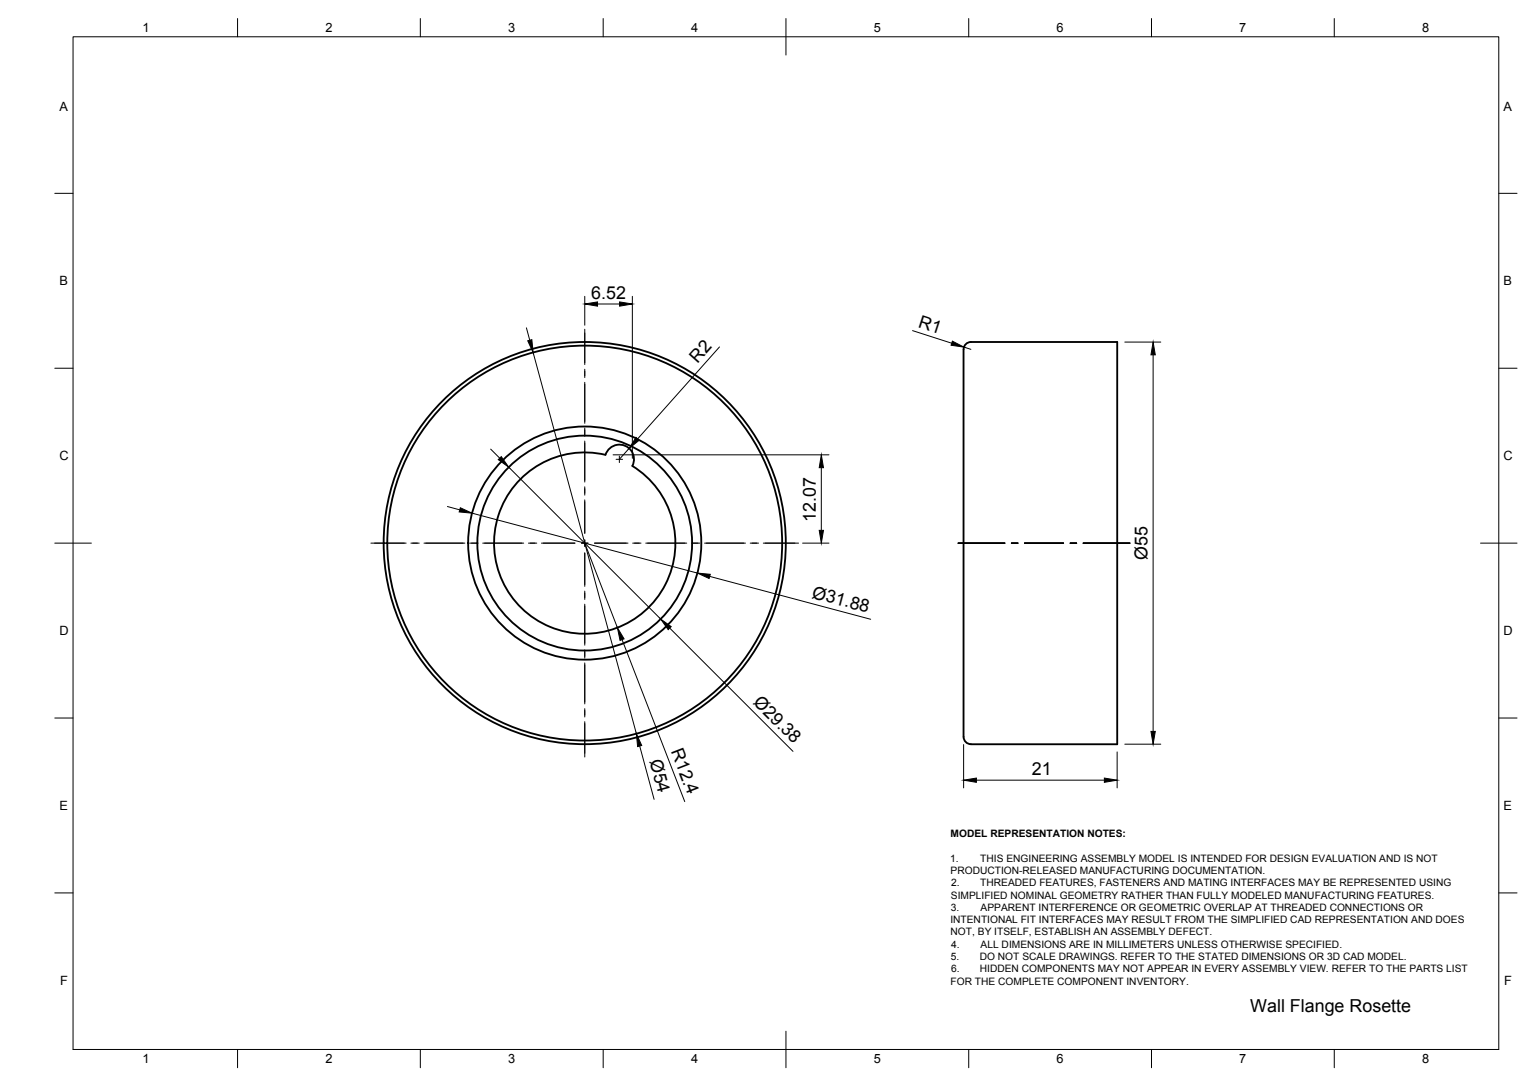
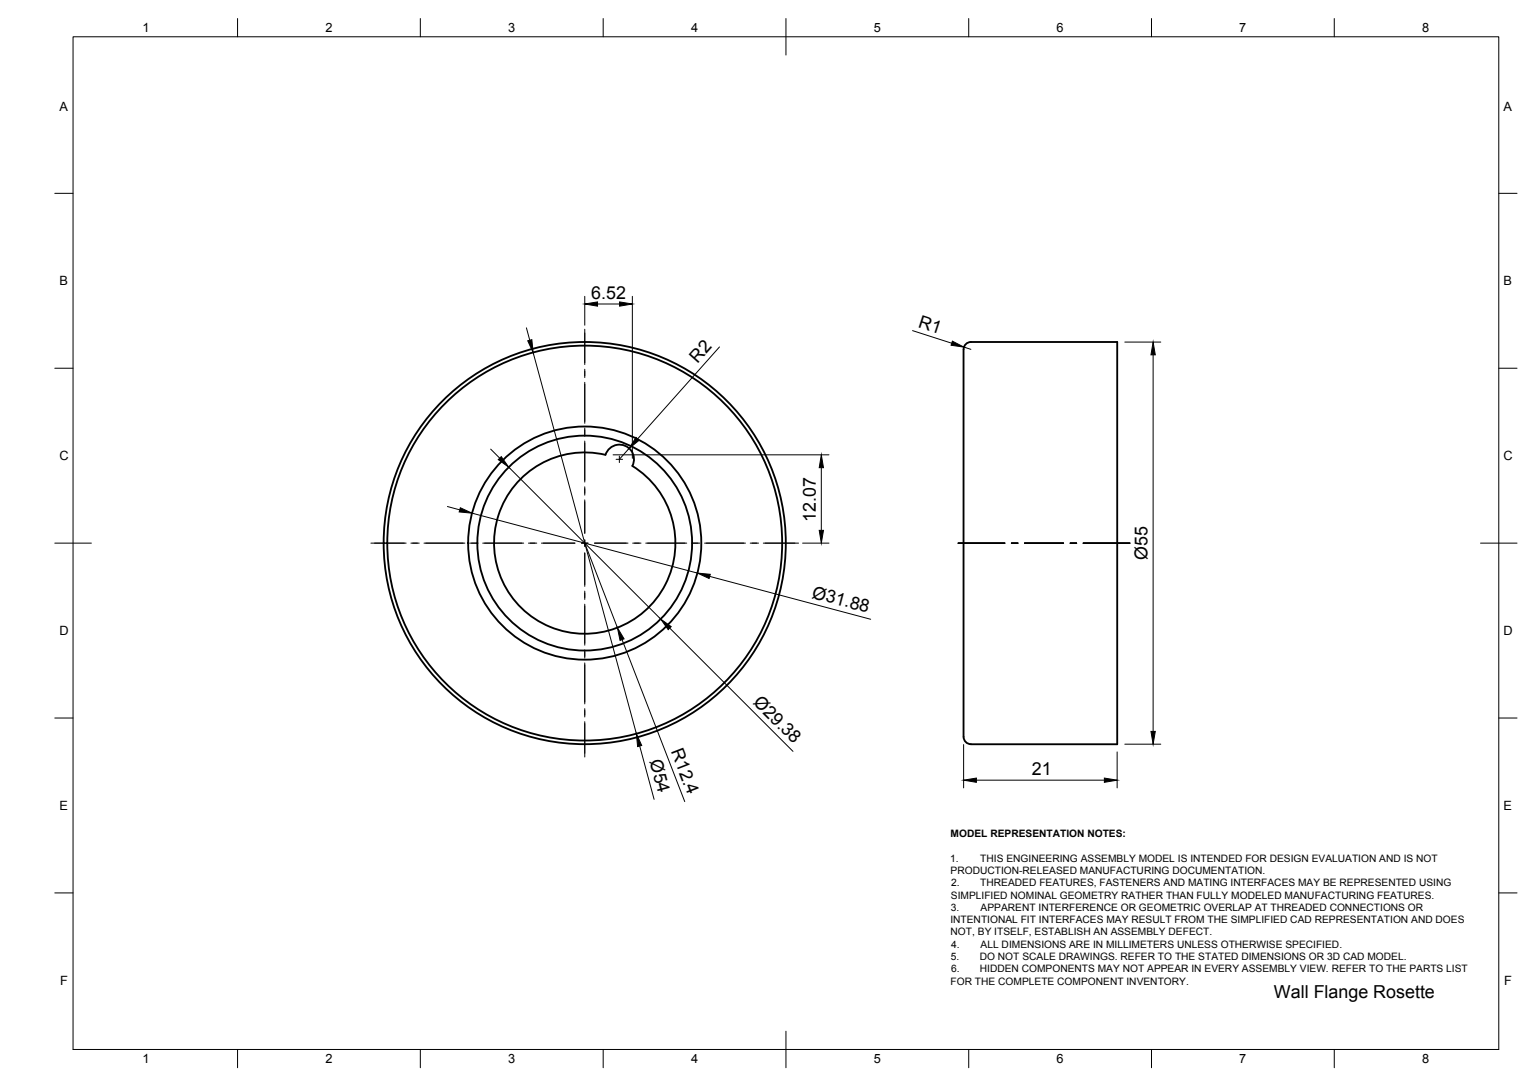
ISO-10303-21;
HEADER;
/* Generated by software containing ST-Developer
 * from STEP Tools, Inc. (www.steptools.com) 
 */

FILE_DESCRIPTION(
/* description */ ('STEP AP214'),
/* implementation_level */ '2;1');

FILE_NAME(
/* name */ 'Wall Flange Rosette.step',
/* time_stamp */ '2026-10-05T23:18:41-07:00',
/* author */ (''),
/* organization */ (''),
/* preprocessor_version */ 'ST-DEVELOPER v20.2',
/* originating_system */ 'Autodesk Translation Framework v15.15.0.0',
/* authorisation */ '');

FILE_SCHEMA (('AUTOMOTIVE_DESIGN { 1 0 10303 214 3 1 1 }'));
ENDSEC;

DATA;
#10=MECHANICAL_DESIGN_GEOMETRIC_PRESENTATION_REPRESENTATION('',(#106),#221662);
#68=MANIFOLD_SOLID_BREP('Body1',#79328);
#80=SHAPE_REPRESENTATION_RELATIONSHIP('SRR','None',#221715,#93);
#93=ADVANCED_BREP_SHAPE_REPRESENTATION('',(#68),#221655);
#106=STYLED_ITEM('',(#221783),#68);
#297=FACE_BOUND('',#24816,.T.);
#298=FACE_BOUND('',#24818,.T.);
#299=FACE_BOUND('',#24820,.T.);
#300=FACE_BOUND('',#24823,.T.);
#301=FACE_BOUND('',#24825,.T.);
#1896=TOROIDAL_SURFACE('',#80767,26.5,1.);
#1897=TOROIDAL_SURFACE('',#80779,26.5,0.5);
#1942=CONICAL_SURFACE('',#80785,15.31367390024,0.849141474959914);
#1943=CONICAL_SURFACE('',#80792,15.125,0.849141474959914);
#2233=CYLINDRICAL_SURFACE('',#80771,27.5);
#2234=CYLINDRICAL_SURFACE('',#80773,12.4);
#2235=CYLINDRICAL_SURFACE('',#80776,2.00000000000001);
#2236=CYLINDRICAL_SURFACE('',#80783,27.);
#3153=LINE('',#177954,#10220);
#3154=LINE('',#177961,#10221);
#3155=LINE('',#177964,#10222);
#3156=LINE('',#177977,#10223);
#3157=LINE('',#177982,#10224);
#3158=LINE('',#177991,#10225);
#10220=VECTOR('',#89196,27.5);
#10221=VECTOR('',#89203,1000.);
#10222=VECTOR('',#89206,1000.);
#10223=VECTOR('',#89225,27.);
#10224=VECTOR('',#89230,15.31367390024);
#10225=VECTOR('',#89243,15.125);
#16989=PLANE('',#80788);
#16990=PLANE('',#80789);
#16991=PLANE('',#80790);
#16992=PLANE('',#80794);
#16993=PLANE('',#80795);
#20741=FACE_OUTER_BOUND('',#24808,.T.);
#20742=FACE_OUTER_BOUND('',#24809,.T.);
#20743=FACE_OUTER_BOUND('',#24810,.T.);
#20744=FACE_OUTER_BOUND('',#24811,.T.);
#20745=FACE_OUTER_BOUND('',#24812,.T.);
#20746=FACE_OUTER_BOUND('',#24813,.T.);
#20747=FACE_OUTER_BOUND('',#24814,.T.);
#20748=FACE_OUTER_BOUND('',#24815,.T.);
#20749=FACE_OUTER_BOUND('',#24817,.T.);
#20750=FACE_OUTER_BOUND('',#24819,.T.);
#20751=FACE_OUTER_BOUND('',#24821,.T.);
#20752=FACE_OUTER_BOUND('',#24822,.T.);
#20753=FACE_OUTER_BOUND('',#24824,.T.);
#24808=EDGE_LOOP('',(#56653,#56654,#56655,#56656));
#24809=EDGE_LOOP('',(#56657,#56658,#56659,#56660));
#24810=EDGE_LOOP('',(#56661,#56662,#56663,#56664));
#24811=EDGE_LOOP('',(#56665,#56666,#56667,#56668));
#24812=EDGE_LOOP('',(#56669,#56670,#56671,#56672));
#24813=EDGE_LOOP('',(#56673,#56674,#56675,#56676));
#24814=EDGE_LOOP('',(#56677,#56678,#56679,#56680));
#24815=EDGE_LOOP('',(#56681));
#24816=EDGE_LOOP('',(#56682));
#24817=EDGE_LOOP('',(#56683));
#24818=EDGE_LOOP('',(#56684,#56685));
#24819=EDGE_LOOP('',(#56686));
#24820=EDGE_LOOP('',(#56687,#56688));
#24821=EDGE_LOOP('',(#56689,#56690,#56691,#56692));
#24822=EDGE_LOOP('',(#56693));
#24823=EDGE_LOOP('',(#56694));
#24824=EDGE_LOOP('',(#56695));
#24825=EDGE_LOOP('',(#56696));
#31299=CIRCLE('',#80768,26.49999955823);
#31300=CIRCLE('',#80769,1.);
#31301=CIRCLE('',#80770,27.5);
#31302=CIRCLE('',#80772,27.5);
#31303=CIRCLE('',#80774,12.4);
#31304=CIRCLE('',#80775,12.4);
#31305=CIRCLE('',#80777,2.);
#31306=CIRCLE('',#80778,2.);
#31307=CIRCLE('',#80780,27.);
#31308=CIRCLE('',#80781,0.5);
#31309=CIRCLE('',#80782,26.5);
#31310=CIRCLE('',#80784,27.);
#31311=CIRCLE('',#80786,15.93867390024);
#31312=CIRCLE('',#80787,14.68867390024);
#31313=CIRCLE('',#80791,14.5);
#31314=CIRCLE('',#80793,15.75);
#34858=VERTEX_POINT('',#177947);
#34859=VERTEX_POINT('',#177949);
#34860=VERTEX_POINT('',#177953);
#34861=VERTEX_POINT('',#177957);
#34862=VERTEX_POINT('',#177958);
#34863=VERTEX_POINT('',#177960);
#34864=VERTEX_POINT('',#177962);
#34865=VERTEX_POINT('',#177969);
#34866=VERTEX_POINT('',#177971);
#34867=VERTEX_POINT('',#177975);
#34868=VERTEX_POINT('',#177979);
#34869=VERTEX_POINT('',#177981);
#34870=VERTEX_POINT('',#177987);
#34871=VERTEX_POINT('',#177990);
#43159=EDGE_CURVE('',#34858,#34858,#31299,.T.);
#43160=EDGE_CURVE('',#34858,#34859,#31300,.T.);
#43161=EDGE_CURVE('',#34859,#34859,#31301,.T.);
#43162=EDGE_CURVE('',#34859,#34860,#3153,.T.);
#43163=EDGE_CURVE('',#34860,#34860,#31302,.T.);
#43164=EDGE_CURVE('',#34861,#34862,#31303,.T.);
#43165=EDGE_CURVE('',#34863,#34861,#3154,.T.);
#43166=EDGE_CURVE('',#34863,#34864,#31304,.T.);
#43167=EDGE_CURVE('',#34864,#34862,#3155,.T.);
#43168=EDGE_CURVE('',#34862,#34861,#31305,.T.);
#43169=EDGE_CURVE('',#34864,#34863,#31306,.T.);
#43170=EDGE_CURVE('',#34865,#34865,#31307,.T.);
#43171=EDGE_CURVE('',#34865,#34866,#31308,.T.);
#43172=EDGE_CURVE('',#34866,#34866,#31309,.T.);
#43173=EDGE_CURVE('',#34867,#34867,#31310,.T.);
#43174=EDGE_CURVE('',#34867,#34865,#3156,.T.);
#43175=EDGE_CURVE('',#34868,#34868,#31311,.T.);
#43176=EDGE_CURVE('',#34868,#34869,#3157,.T.);
#43177=EDGE_CURVE('',#34869,#34869,#31312,.T.);
#43178=EDGE_CURVE('',#34870,#34870,#31313,.T.);
#43179=EDGE_CURVE('',#34870,#34871,#3158,.T.);
#43180=EDGE_CURVE('',#34871,#34871,#31314,.T.);
#56653=ORIENTED_EDGE('',*,*,#43159,.F.);
#56654=ORIENTED_EDGE('',*,*,#43160,.T.);
#56655=ORIENTED_EDGE('',*,*,#43161,.T.);
#56656=ORIENTED_EDGE('',*,*,#43160,.F.);
#56657=ORIENTED_EDGE('',*,*,#43161,.F.);
#56658=ORIENTED_EDGE('',*,*,#43162,.T.);
#56659=ORIENTED_EDGE('',*,*,#43163,.T.);
#56660=ORIENTED_EDGE('',*,*,#43162,.F.);
#56661=ORIENTED_EDGE('',*,*,#43164,.F.);
#56662=ORIENTED_EDGE('',*,*,#43165,.F.);
#56663=ORIENTED_EDGE('',*,*,#43166,.T.);
#56664=ORIENTED_EDGE('',*,*,#43167,.T.);
#56665=ORIENTED_EDGE('',*,*,#43168,.F.);
#56666=ORIENTED_EDGE('',*,*,#43167,.F.);
#56667=ORIENTED_EDGE('',*,*,#43169,.T.);
#56668=ORIENTED_EDGE('',*,*,#43165,.T.);
#56669=ORIENTED_EDGE('',*,*,#43170,.F.);
#56670=ORIENTED_EDGE('',*,*,#43171,.T.);
#56671=ORIENTED_EDGE('',*,*,#43172,.T.);
#56672=ORIENTED_EDGE('',*,*,#43171,.F.);
#56673=ORIENTED_EDGE('',*,*,#43173,.F.);
#56674=ORIENTED_EDGE('',*,*,#43174,.T.);
#56675=ORIENTED_EDGE('',*,*,#43170,.T.);
#56676=ORIENTED_EDGE('',*,*,#43174,.F.);
#56677=ORIENTED_EDGE('',*,*,#43175,.F.);
#56678=ORIENTED_EDGE('',*,*,#43176,.T.);
#56679=ORIENTED_EDGE('',*,*,#43177,.T.);
#56680=ORIENTED_EDGE('',*,*,#43176,.F.);
#56681=ORIENTED_EDGE('',*,*,#43172,.F.);
#56682=ORIENTED_EDGE('',*,*,#43175,.T.);
#56683=ORIENTED_EDGE('',*,*,#43177,.F.);
#56684=ORIENTED_EDGE('',*,*,#43169,.F.);
#56685=ORIENTED_EDGE('',*,*,#43166,.F.);
#56686=ORIENTED_EDGE('',*,*,#43178,.T.);
#56687=ORIENTED_EDGE('',*,*,#43168,.T.);
#56688=ORIENTED_EDGE('',*,*,#43164,.T.);
#56689=ORIENTED_EDGE('',*,*,#43178,.F.);
#56690=ORIENTED_EDGE('',*,*,#43179,.T.);
#56691=ORIENTED_EDGE('',*,*,#43180,.T.);
#56692=ORIENTED_EDGE('',*,*,#43179,.F.);
#56693=ORIENTED_EDGE('',*,*,#43159,.T.);
#56694=ORIENTED_EDGE('',*,*,#43180,.F.);
#56695=ORIENTED_EDGE('',*,*,#43163,.F.);
#56696=ORIENTED_EDGE('',*,*,#43173,.T.);
#76171=ADVANCED_FACE('',(#20741),#1896,.T.);
#76172=ADVANCED_FACE('',(#20742),#2233,.T.);
#76173=ADVANCED_FACE('',(#20743),#2234,.F.);
#76174=ADVANCED_FACE('',(#20744),#2235,.F.);
#76175=ADVANCED_FACE('',(#20745),#1897,.F.);
#76176=ADVANCED_FACE('',(#20746),#2236,.F.);
#76177=ADVANCED_FACE('',(#20747),#1942,.T.);
#76178=ADVANCED_FACE('',(#20748,#297),#16989,.F.);
#76179=ADVANCED_FACE('',(#20749,#298),#16990,.F.);
#76180=ADVANCED_FACE('',(#20750,#299),#16991,.T.);
#76181=ADVANCED_FACE('',(#20751),#1943,.F.);
#76182=ADVANCED_FACE('',(#20752,#300),#16992,.T.);
#76183=ADVANCED_FACE('',(#20753,#301),#16993,.F.);
#79328=CLOSED_SHELL('',(#76171,#76172,#76173,#76174,#76175,#76176,#76177,
#76178,#76179,#76180,#76181,#76182,#76183));
#80766=AXIS2_PLACEMENT_3D('',#177945,#89184,#89185);
#80767=AXIS2_PLACEMENT_3D('',#177946,#89186,#89187);
#80768=AXIS2_PLACEMENT_3D('',#177948,#89188,#89189);
#80769=AXIS2_PLACEMENT_3D('',#177950,#89190,#89191);
#80770=AXIS2_PLACEMENT_3D('',#177951,#89192,#89193);
#80771=AXIS2_PLACEMENT_3D('',#177952,#89194,#89195);
#80772=AXIS2_PLACEMENT_3D('',#177955,#89197,#89198);
#80773=AXIS2_PLACEMENT_3D('',#177956,#89199,#89200);
#80774=AXIS2_PLACEMENT_3D('',#177959,#89201,#89202);
#80775=AXIS2_PLACEMENT_3D('',#177963,#89204,#89205);
#80776=AXIS2_PLACEMENT_3D('',#177965,#89207,#89208);
#80777=AXIS2_PLACEMENT_3D('',#177966,#89209,#89210);
#80778=AXIS2_PLACEMENT_3D('',#177967,#89211,#89212);
#80779=AXIS2_PLACEMENT_3D('',#177968,#89213,#89214);
#80780=AXIS2_PLACEMENT_3D('',#177970,#89215,#89216);
#80781=AXIS2_PLACEMENT_3D('',#177972,#89217,#89218);
#80782=AXIS2_PLACEMENT_3D('',#177973,#89219,#89220);
#80783=AXIS2_PLACEMENT_3D('',#177974,#89221,#89222);
#80784=AXIS2_PLACEMENT_3D('',#177976,#89223,#89224);
#80785=AXIS2_PLACEMENT_3D('',#177978,#89226,#89227);
#80786=AXIS2_PLACEMENT_3D('',#177980,#89228,#89229);
#80787=AXIS2_PLACEMENT_3D('',#177983,#89231,#89232);
#80788=AXIS2_PLACEMENT_3D('',#177984,#89233,#89234);
#80789=AXIS2_PLACEMENT_3D('',#177985,#89235,#89236);
#80790=AXIS2_PLACEMENT_3D('',#177986,#89237,#89238);
#80791=AXIS2_PLACEMENT_3D('',#177988,#89239,#89240);
#80792=AXIS2_PLACEMENT_3D('',#177989,#89241,#89242);
#80793=AXIS2_PLACEMENT_3D('',#177992,#89244,#89245);
#80794=AXIS2_PLACEMENT_3D('',#177993,#89246,#89247);
#80795=AXIS2_PLACEMENT_3D('',#177994,#89248,#89249);
#89184=DIRECTION('axis',(0.,0.,1.));
#89185=DIRECTION('refdir',(1.,0.,0.));
#89186=DIRECTION('center_axis',(1.,0.,0.));
#89187=DIRECTION('ref_axis',(0.,0.924224592736303,0.381849318686593));
#89188=DIRECTION('center_axis',(1.,0.,0.));
#89189=DIRECTION('ref_axis',(0.,0.381849318686592,-0.924224592736303));
#89190=DIRECTION('center_axis',(0.,0.381849318686593,-0.924224592736303));
#89191=DIRECTION('ref_axis',(0.,-0.924224592736303,-0.381849318686593));
#89192=DIRECTION('center_axis',(1.,0.,0.));
#89193=DIRECTION('ref_axis',(0.,0.381849318686593,-0.924224592736303));
#89194=DIRECTION('center_axis',(1.,0.,0.));
#89195=DIRECTION('ref_axis',(0.,0.924224592736303,0.381849318686593));
#89196=DIRECTION('',(-1.,0.,0.));
#89197=DIRECTION('center_axis',(1.,0.,0.));
#89198=DIRECTION('ref_axis',(0.,0.381849318686593,-0.924224592736303));
#89199=DIRECTION('center_axis',(-1.,0.,0.));
#89200=DIRECTION('ref_axis',(0.,0.381849318686589,-0.924224592736304));
#89201=DIRECTION('center_axis',(-1.,0.,0.));
#89202=DIRECTION('ref_axis',(0.,-0.228299548172813,0.973590938897897));
#89203=DIRECTION('',(1.,0.,0.));
#89204=DIRECTION('center_axis',(-1.,0.,0.));
#89205=DIRECTION('ref_axis',(0.,-0.228299548172813,0.973590938897897));
#89206=DIRECTION('',(1.,0.,0.));
#89207=DIRECTION('center_axis',(-1.,0.,0.));
#89208=DIRECTION('ref_axis',(0.,-0.381849318686606,0.924224592736298));
#89209=DIRECTION('center_axis',(-1.,0.,0.));
#89210=DIRECTION('ref_axis',(0.,-0.890419977397047,-0.455139828901232));
#89211=DIRECTION('center_axis',(-1.,0.,0.));
#89212=DIRECTION('ref_axis',(0.,-0.890419977397047,-0.455139828901232));
#89213=DIRECTION('center_axis',(1.,0.,0.));
#89214=DIRECTION('ref_axis',(0.,0.924224592736303,0.381849318686593));
#89215=DIRECTION('center_axis',(1.,0.,0.));
#89216=DIRECTION('ref_axis',(0.,0.381849318686593,-0.924224592736303));
#89217=DIRECTION('center_axis',(0.,-0.381849318686593,0.924224592736303));
#89218=DIRECTION('ref_axis',(0.,-0.924224592736303,-0.381849318686593));
#89219=DIRECTION('center_axis',(1.,0.,0.));
#89220=DIRECTION('ref_axis',(0.,0.381849318686592,-0.924224592736303));
#89221=DIRECTION('center_axis',(1.,0.,0.));
#89222=DIRECTION('ref_axis',(0.,0.924224592736303,0.381849318686593));
#89223=DIRECTION('center_axis',(1.,0.,0.));
#89224=DIRECTION('ref_axis',(0.,0.381849318686593,-0.924224592736303));
#89225=DIRECTION('',(1.,0.,0.));
#89226=DIRECTION('center_axis',(1.,2.78424187714042E-18,1.15032739033389E-18));
#89227=DIRECTION('ref_axis',(-3.01251654524499E-18,0.924224592736303,0.381849318686592));
#89228=DIRECTION('center_axis',(1.,0.,0.));
#89229=DIRECTION('ref_axis',(0.,-0.924224592736303,-0.381849318686593));
#89230=DIRECTION('',(-0.660627895620383,0.693827893847185,0.286659444721021));
#89231=DIRECTION('center_axis',(1.,0.,0.));
#89232=DIRECTION('ref_axis',(0.,0.924224592736303,0.381849318686593));
#89233=DIRECTION('center_axis',(1.,0.,0.));
#89234=DIRECTION('ref_axis',(0.,1.,0.));
#89235=DIRECTION('center_axis',(1.,0.,0.));
#89236=DIRECTION('ref_axis',(0.,1.,0.));
#89237=DIRECTION('center_axis',(1.,0.,0.));
#89238=DIRECTION('ref_axis',(0.,1.,0.));
#89239=DIRECTION('center_axis',(1.,0.,0.));
#89240=DIRECTION('ref_axis',(0.,0.924224592736303,0.381849318686593));
#89241=DIRECTION('center_axis',(1.,-4.17704712177877E-17,-1.72577381094218E-17));
#89242=DIRECTION('ref_axis',(4.51951522888177E-17,0.924224592736303,0.381849318686593));
#89243=DIRECTION('',(0.660627895620383,-0.693827893847184,-0.286659444721022));
#89244=DIRECTION('center_axis',(1.,0.,0.));
#89245=DIRECTION('ref_axis',(0.,0.924224592736303,0.381849318686592));
#89246=DIRECTION('center_axis',(1.,0.,0.));
#89247=DIRECTION('ref_axis',(0.,1.,0.));
#89248=DIRECTION('center_axis',(1.,0.,0.));
#89249=DIRECTION('ref_axis',(0.,1.,0.));
#177945=CARTESIAN_POINT('',(0.,0.,0.));
#177946=CARTESIAN_POINT('Origin',(-30.5675364832709,75.,72.98888938658));
#177947=CARTESIAN_POINT('',(-29.5675364832709,50.5080487007827,62.8698826100749));
#177948=CARTESIAN_POINT('Origin',(-29.5675364832709,75.,72.98888938658));
#177949=CARTESIAN_POINT('',(-30.5675364832709,49.5838236997517,62.4880331226987));
#177950=CARTESIAN_POINT('Origin',(-30.5675364832709,50.508048292488,62.8698824413853));
#177951=CARTESIAN_POINT('Origin',(-30.5675364832709,75.,72.98888938658));
#177952=CARTESIAN_POINT('Origin',(-50.5675364832709,75.,72.98888938658));
#177953=CARTESIAN_POINT('',(-50.5675364832709,49.5838236997517,62.4880331226987));
#177954=CARTESIAN_POINT('',(-50.5675364832709,49.5838236997517,62.4880331226987));
#177955=CARTESIAN_POINT('Origin',(-50.5675364832709,75.,72.98888938658));
#177956=CARTESIAN_POINT('Origin',(-50.5675364832709,75.,72.98888938658));
#177957=CARTESIAN_POINT('',(-30.6675364832709,72.1690856026562,85.0614170289144));
#177958=CARTESIAN_POINT('',(-30.6675364832709,68.4842284934922,83.5389946787084));
#177959=CARTESIAN_POINT('Origin',(-30.6675364832709,75.,72.98888938658));
#177960=CARTESIAN_POINT('',(-31.1675364832709,72.1690856026562,85.0614170289144));
#177961=CARTESIAN_POINT('',(-31.1675364832709,72.1690856026562,85.0614170289144));
#177962=CARTESIAN_POINT('',(-31.1675364832709,68.4842284934922,83.5389946787084));
#177963=CARTESIAN_POINT('Origin',(-31.1675364832709,75.,72.98888938658));
#177964=CARTESIAN_POINT('',(-31.1675364832709,68.4842284934922,83.5389946787084));
#177965=CARTESIAN_POINT('Origin',(-50.5675364832709,70.2650684482863,84.4492743365102));
#177966=CARTESIAN_POINT('Origin',(-30.6675364832709,70.2650684482863,84.4492743365102));
#177967=CARTESIAN_POINT('Origin',(-31.1675364832709,70.2650684482863,84.4492743365102));
#177968=CARTESIAN_POINT('Origin',(-30.5675364832709,75.,72.98888938658));
#177969=CARTESIAN_POINT('',(-30.5675364832709,50.0459359961198,62.678957782042));
#177970=CARTESIAN_POINT('Origin',(-30.5675364832709,75.,72.98888938658));
#177971=CARTESIAN_POINT('',(-30.0675364832709,50.508048292488,62.8698824413853));
#177972=CARTESIAN_POINT('Origin',(-30.5675364832709,50.508048292488,62.8698824413853));
#177973=CARTESIAN_POINT('Origin',(-30.0675364832709,75.,72.98888938658));
#177974=CARTESIAN_POINT('Origin',(-50.5675364832709,75.,72.98888938658));
#177975=CARTESIAN_POINT('',(-50.5675364832709,50.0459359961198,62.678957782042));
#177976=CARTESIAN_POINT('Origin',(-50.5675364832709,75.,72.98888938658));
#177977=CARTESIAN_POINT('',(-50.5675364832709,50.0459359961198,62.678957782042));
#177978=CARTESIAN_POINT('Origin',(-30.6175364832709,75.,72.98888938658));
#177979=CARTESIAN_POINT('',(-30.0675364832709,60.269085605794,66.9027176170056));
#177980=CARTESIAN_POINT('Origin',(-30.0675364832709,75.,72.98888938658));
#177981=CARTESIAN_POINT('',(-31.1675364832709,61.4243663467144,67.3800292653639));
#177982=CARTESIAN_POINT('',(-30.6175364832709,60.8467259762541,67.1413734411847));
#177983=CARTESIAN_POINT('Origin',(-31.1675364832709,75.,72.98888938658));
#177984=CARTESIAN_POINT('Origin',(-30.0675364832709,75.,72.98888938658));
#177985=CARTESIAN_POINT('Origin',(-31.1675364832709,75.,72.98888938658));
#177986=CARTESIAN_POINT('Origin',(-30.6675364832709,75.,72.98888938658));
#177987=CARTESIAN_POINT('',(-30.6675364832709,61.5987434053236,67.4520742656245));
#177988=CARTESIAN_POINT('Origin',(-30.6675364832709,75.,72.98888938658));
#177989=CARTESIAN_POINT('Origin',(-30.1175364832709,75.,72.98888938658));
#177990=CARTESIAN_POINT('',(-29.5675364832709,60.4434626644033,66.9747626172662));
#177991=CARTESIAN_POINT('',(-30.1175364832709,61.0211030348634,67.2134184414453));
#177992=CARTESIAN_POINT('Origin',(-29.5675364832709,75.,72.98888938658));
#177993=CARTESIAN_POINT('Origin',(-29.5675364832709,75.,72.98888938658));
#177994=CARTESIAN_POINT('Origin',(-50.5675364832709,75.,72.98888938658));
#221640=UNCERTAINTY_MEASURE_WITH_UNIT(LENGTH_MEASURE(0.01),#221663,
'DISTANCE_ACCURACY_VALUE',
'Maximum model space distance between geometric entities at asserted c
onnectivities');
#221647=UNCERTAINTY_MEASURE_WITH_UNIT(LENGTH_MEASURE(0.01),#221663,
'DISTANCE_ACCURACY_VALUE',
'Maximum model space distance between geometric entities at asserted c
onnectivities');
#221655=(
GEOMETRIC_REPRESENTATION_CONTEXT(3)
GLOBAL_UNCERTAINTY_ASSIGNED_CONTEXT((#221640))
GLOBAL_UNIT_ASSIGNED_CONTEXT((#221663,#221665,#221666))
REPRESENTATION_CONTEXT('','3D')
);
#221662=(
GEOMETRIC_REPRESENTATION_CONTEXT(3)
GLOBAL_UNCERTAINTY_ASSIGNED_CONTEXT((#221647))
GLOBAL_UNIT_ASSIGNED_CONTEXT((#221663,#221665,#221666))
REPRESENTATION_CONTEXT('','3D')
);
#221663=(
LENGTH_UNIT()
NAMED_UNIT(*)
SI_UNIT(.MILLI.,.METRE.)
);
#221665=(
NAMED_UNIT(*)
PLANE_ANGLE_UNIT()
SI_UNIT($,.RADIAN.)
);
#221666=(
NAMED_UNIT(*)
SI_UNIT($,.STERADIAN.)
SOLID_ANGLE_UNIT()
);
#221674=SHAPE_DEFINITION_REPRESENTATION(#221688,#221715);
#221688=PRODUCT_DEFINITION_SHAPE('',$,#221730);
#221715=SHAPE_REPRESENTATION('',(#80766),#221655);
#221722=PRODUCT_DEFINITION_CONTEXT('part definition',#221766,'design');
#221730=PRODUCT_DEFINITION('2026-10-05-23-02-39-335',
'Wall Flange Rosette',#221744,#221722);
#221744=PRODUCT_DEFINITION_FORMATION('',$,#221775);
#221766=APPLICATION_CONTEXT(
'Core Data for Automotive Mechanical Design Process');
#221767=PRODUCT_CONTEXT('part definition',#221766,'mechanical');
#221775=PRODUCT('2026-10-05-23-02-39-335','Wall Flange Rosette',$,(#221767));
#221783=PRESENTATION_STYLE_ASSIGNMENT((#221785));
#221785=SURFACE_STYLE_USAGE(.BOTH.,#221787);
#221787=SURFACE_SIDE_STYLE('',(#221789));
#221789=SURFACE_STYLE_FILL_AREA(#221791);
#221791=FILL_AREA_STYLE('Opaque(202,209,238)',(#221793));
#221793=FILL_AREA_STYLE_COLOUR('Opaque(202,209,238)',#221795);
#221795=COLOUR_RGB('Opaque(202,209,238)', 0.09019608, 0.27058824, 0.51372549);
ENDSEC;
END-ISO-10303-21;
